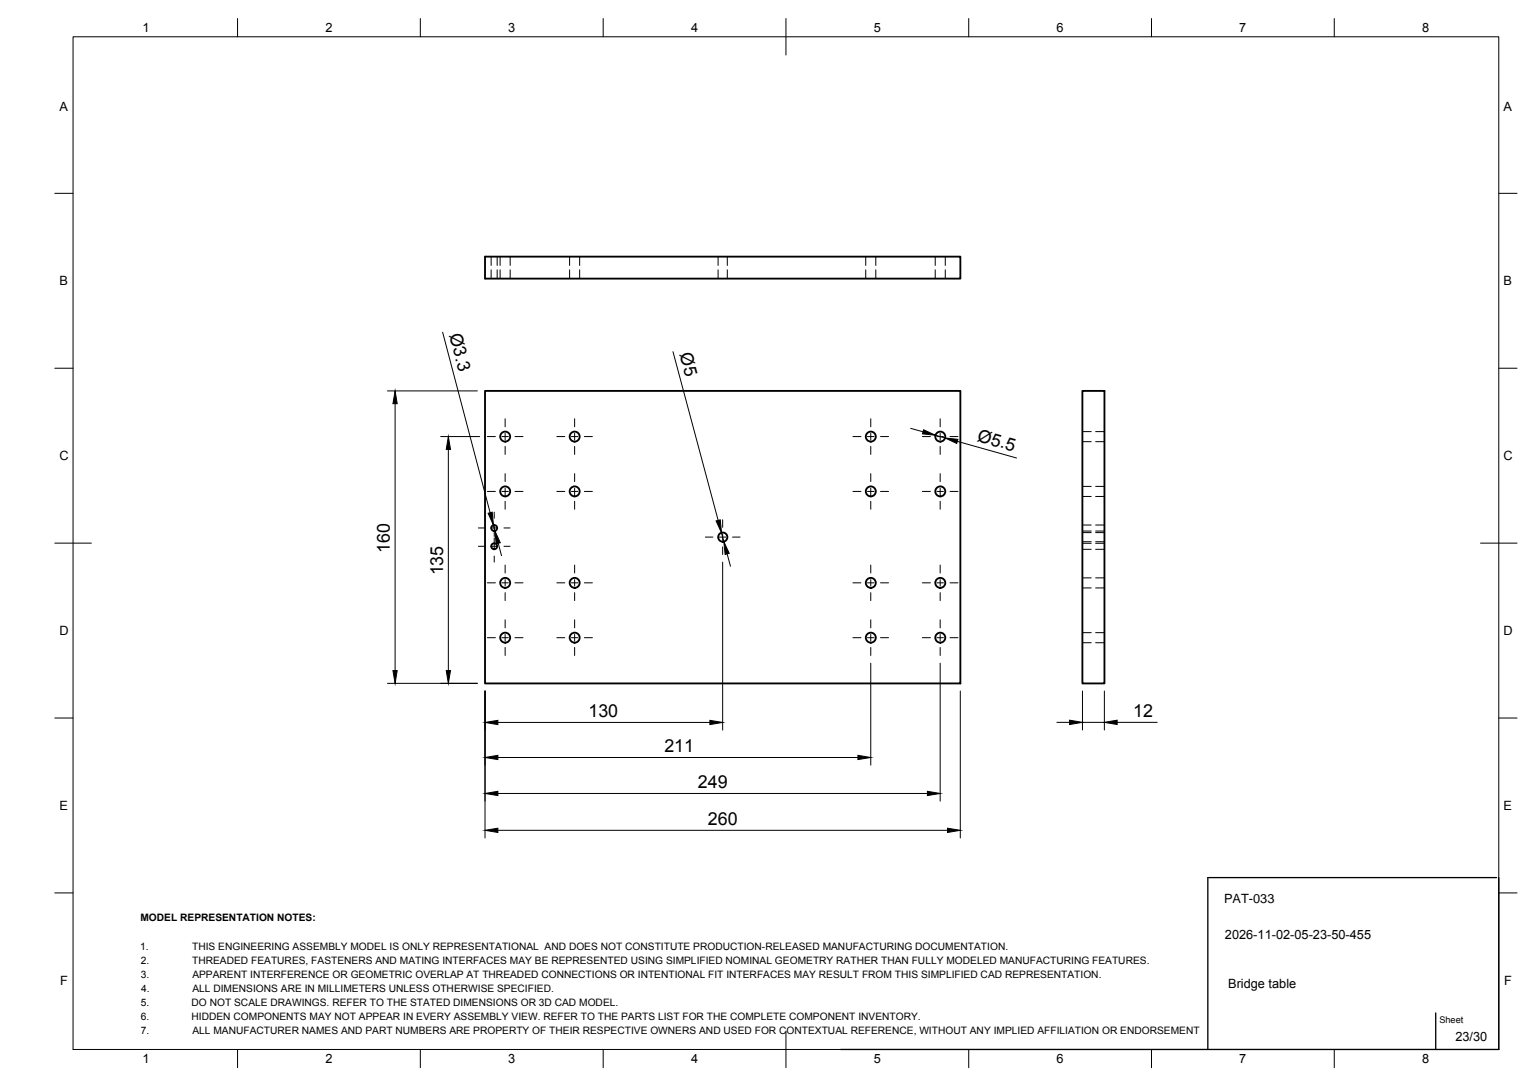
ISO-10303-21;
HEADER;
/* Generated by software containing ST-Developer
 * from STEP Tools, Inc. (www.steptools.com) 
 */

FILE_DESCRIPTION(
/* description */ ('Dual-rail gantry carriage'),
/* implementation_level */ '2;1');

FILE_NAME(
/* name */ 'Bridge table.step',
/* time_stamp */ '2026-10-27T10:49:15-07:00',
/* author */ (''),
/* organization */ (''),
/* preprocessor_version */ 'ST-DEVELOPER v20.2',
/* originating_system */ 'Autodesk Translation Framework v15.17.0.0',
/* authorisation */ '');

FILE_SCHEMA (('AUTOMOTIVE_DESIGN { 1 0 10303 214 3 1 1 }'));
ENDSEC;

DATA;
#10=MECHANICAL_DESIGN_GEOMETRIC_PRESENTATION_REPRESENTATION('',(#604),#12804);
#542=SHAPE_REPRESENTATION_RELATIONSHIP('SRR','None',#13021,#573);
#573=ADVANCED_BREP_SHAPE_REPRESENTATION('',(#633),#12791);
#604=STYLED_ITEM('',(#13233),#633);
#633=MANIFOLD_SOLID_BREP('Body1',#7384);
#707=FACE_BOUND('',#1770,.T.);
#708=FACE_BOUND('',#1771,.T.);
#709=FACE_BOUND('',#1772,.T.);
#710=FACE_BOUND('',#1773,.T.);
#711=FACE_BOUND('',#1774,.T.);
#712=FACE_BOUND('',#1775,.T.);
#713=FACE_BOUND('',#1776,.T.);
#714=FACE_BOUND('',#1777,.T.);
#715=FACE_BOUND('',#1778,.T.);
#716=FACE_BOUND('',#1779,.T.);
#717=FACE_BOUND('',#1780,.T.);
#718=FACE_BOUND('',#1781,.T.);
#719=FACE_BOUND('',#1782,.T.);
#720=FACE_BOUND('',#1783,.T.);
#721=FACE_BOUND('',#1784,.T.);
#722=FACE_BOUND('',#1785,.T.);
#723=FACE_BOUND('',#1786,.T.);
#724=FACE_BOUND('',#1787,.T.);
#725=FACE_BOUND('',#1788,.T.);
#726=FACE_BOUND('',#1790,.T.);
#727=FACE_BOUND('',#1791,.T.);
#728=FACE_BOUND('',#1792,.T.);
#729=FACE_BOUND('',#1793,.T.);
#730=FACE_BOUND('',#1794,.T.);
#731=FACE_BOUND('',#1795,.T.);
#732=FACE_BOUND('',#1796,.T.);
#733=FACE_BOUND('',#1797,.T.);
#734=FACE_BOUND('',#1798,.T.);
#735=FACE_BOUND('',#1799,.T.);
#736=FACE_BOUND('',#1800,.T.);
#737=FACE_BOUND('',#1801,.T.);
#738=FACE_BOUND('',#1802,.T.);
#739=FACE_BOUND('',#1803,.T.);
#740=FACE_BOUND('',#1804,.T.);
#741=FACE_BOUND('',#1805,.T.);
#742=FACE_BOUND('',#1806,.T.);
#743=FACE_BOUND('',#1807,.T.);
#744=FACE_BOUND('',#1808,.T.);
#955=PLANE('',#8168);
#956=PLANE('',#8169);
#957=PLANE('',#8170);
#958=PLANE('',#8171);
#959=PLANE('',#8172);
#960=PLANE('',#8173);
#1292=FACE_OUTER_BOUND('',#1746,.T.);
#1293=FACE_OUTER_BOUND('',#1747,.T.);
#1294=FACE_OUTER_BOUND('',#1748,.T.);
#1295=FACE_OUTER_BOUND('',#1749,.T.);
#1296=FACE_OUTER_BOUND('',#1750,.T.);
#1297=FACE_OUTER_BOUND('',#1751,.T.);
#1298=FACE_OUTER_BOUND('',#1752,.T.);
#1299=FACE_OUTER_BOUND('',#1753,.T.);
#1300=FACE_OUTER_BOUND('',#1754,.T.);
#1301=FACE_OUTER_BOUND('',#1755,.T.);
#1302=FACE_OUTER_BOUND('',#1756,.T.);
#1303=FACE_OUTER_BOUND('',#1757,.T.);
#1304=FACE_OUTER_BOUND('',#1758,.T.);
#1305=FACE_OUTER_BOUND('',#1759,.T.);
#1306=FACE_OUTER_BOUND('',#1760,.T.);
#1307=FACE_OUTER_BOUND('',#1761,.T.);
#1308=FACE_OUTER_BOUND('',#1762,.T.);
#1309=FACE_OUTER_BOUND('',#1763,.T.);
#1310=FACE_OUTER_BOUND('',#1764,.T.);
#1311=FACE_OUTER_BOUND('',#1765,.T.);
#1312=FACE_OUTER_BOUND('',#1766,.T.);
#1313=FACE_OUTER_BOUND('',#1767,.T.);
#1314=FACE_OUTER_BOUND('',#1768,.T.);
#1315=FACE_OUTER_BOUND('',#1769,.T.);
#1316=FACE_OUTER_BOUND('',#1789,.T.);
#1746=EDGE_LOOP('',(#6219,#6220,#6221,#6222));
#1747=EDGE_LOOP('',(#6223,#6224,#6225,#6226));
#1748=EDGE_LOOP('',(#6227,#6228,#6229,#6230));
#1749=EDGE_LOOP('',(#6231,#6232,#6233,#6234));
#1750=EDGE_LOOP('',(#6235,#6236,#6237,#6238));
#1751=EDGE_LOOP('',(#6239,#6240,#6241,#6242));
#1752=EDGE_LOOP('',(#6243,#6244,#6245,#6246));
#1753=EDGE_LOOP('',(#6247,#6248,#6249,#6250));
#1754=EDGE_LOOP('',(#6251,#6252,#6253,#6254));
#1755=EDGE_LOOP('',(#6255,#6256,#6257,#6258));
#1756=EDGE_LOOP('',(#6259,#6260,#6261,#6262));
#1757=EDGE_LOOP('',(#6263,#6264,#6265,#6266));
#1758=EDGE_LOOP('',(#6267,#6268,#6269,#6270));
#1759=EDGE_LOOP('',(#6271,#6272,#6273,#6274));
#1760=EDGE_LOOP('',(#6275,#6276,#6277,#6278));
#1761=EDGE_LOOP('',(#6279,#6280,#6281,#6282));
#1762=EDGE_LOOP('',(#6283,#6284,#6285,#6286));
#1763=EDGE_LOOP('',(#6287,#6288,#6289,#6290));
#1764=EDGE_LOOP('',(#6291,#6292,#6293,#6294));
#1765=EDGE_LOOP('',(#6295,#6296,#6297,#6298));
#1766=EDGE_LOOP('',(#6299,#6300,#6301,#6302));
#1767=EDGE_LOOP('',(#6303,#6304,#6305,#6306));
#1768=EDGE_LOOP('',(#6307,#6308,#6309,#6310));
#1769=EDGE_LOOP('',(#6311,#6312,#6313,#6314));
#1770=EDGE_LOOP('',(#6315));
#1771=EDGE_LOOP('',(#6316));
#1772=EDGE_LOOP('',(#6317));
#1773=EDGE_LOOP('',(#6318));
#1774=EDGE_LOOP('',(#6319));
#1775=EDGE_LOOP('',(#6320));
#1776=EDGE_LOOP('',(#6321));
#1777=EDGE_LOOP('',(#6322));
#1778=EDGE_LOOP('',(#6323));
#1779=EDGE_LOOP('',(#6324));
#1780=EDGE_LOOP('',(#6325));
#1781=EDGE_LOOP('',(#6326));
#1782=EDGE_LOOP('',(#6327));
#1783=EDGE_LOOP('',(#6328));
#1784=EDGE_LOOP('',(#6329));
#1785=EDGE_LOOP('',(#6330));
#1786=EDGE_LOOP('',(#6331));
#1787=EDGE_LOOP('',(#6332));
#1788=EDGE_LOOP('',(#6333));
#1789=EDGE_LOOP('',(#6334,#6335,#6336,#6337));
#1790=EDGE_LOOP('',(#6338));
#1791=EDGE_LOOP('',(#6339));
#1792=EDGE_LOOP('',(#6340));
#1793=EDGE_LOOP('',(#6341));
#1794=EDGE_LOOP('',(#6342));
#1795=EDGE_LOOP('',(#6343));
#1796=EDGE_LOOP('',(#6344));
#1797=EDGE_LOOP('',(#6345));
#1798=EDGE_LOOP('',(#6346));
#1799=EDGE_LOOP('',(#6347));
#1800=EDGE_LOOP('',(#6348));
#1801=EDGE_LOOP('',(#6349));
#1802=EDGE_LOOP('',(#6350));
#1803=EDGE_LOOP('',(#6351));
#1804=EDGE_LOOP('',(#6352));
#1805=EDGE_LOOP('',(#6353));
#1806=EDGE_LOOP('',(#6354));
#1807=EDGE_LOOP('',(#6355));
#1808=EDGE_LOOP('',(#6356));
#2421=LINE('',#11906,#3130);
#2422=LINE('',#11912,#3131);
#2423=LINE('',#11918,#3132);
#2424=LINE('',#11924,#3133);
#2425=LINE('',#11930,#3134);
#2426=LINE('',#11936,#3135);
#2427=LINE('',#11942,#3136);
#2428=LINE('',#11948,#3137);
#2429=LINE('',#11954,#3138);
#2430=LINE('',#11960,#3139);
#2431=LINE('',#11966,#3140);
#2432=LINE('',#11972,#3141);
#2433=LINE('',#11978,#3142);
#2434=LINE('',#11984,#3143);
#2435=LINE('',#11990,#3144);
#2436=LINE('',#11996,#3145);
#2437=LINE('',#12002,#3146);
#2438=LINE('',#12008,#3147);
#2439=LINE('',#12014,#3148);
#2440=LINE('',#12019,#3149);
#2441=LINE('',#12021,#3150);
#2442=LINE('',#12023,#3151);
#2443=LINE('',#12024,#3152);
#2444=LINE('',#12027,#3153);
#2445=LINE('',#12029,#3154);
#2446=LINE('',#12030,#3155);
#2447=LINE('',#12033,#3156);
#2448=LINE('',#12035,#3157);
#2449=LINE('',#12036,#3158);
#2450=LINE('',#12038,#3159);
#2451=LINE('',#12039,#3160);
#3130=VECTOR('',#9704,0.164999999999999);
#3131=VECTOR('',#9711,0.164999999999999);
#3132=VECTOR('',#9718,0.25);
#3133=VECTOR('',#9725,0.274999999999999);
#3134=VECTOR('',#9732,0.274999999999999);
#3135=VECTOR('',#9739,0.274999999999999);
#3136=VECTOR('',#9746,0.274999999999999);
#3137=VECTOR('',#9753,0.274999999999999);
#3138=VECTOR('',#9760,0.275);
#3139=VECTOR('',#9767,0.275);
#3140=VECTOR('',#9774,0.274999999999999);
#3141=VECTOR('',#9781,0.274999999999999);
#3142=VECTOR('',#9788,0.274999999999999);
#3143=VECTOR('',#9795,0.274999999999999);
#3144=VECTOR('',#9802,0.274999999999999);
#3145=VECTOR('',#9809,0.274999999999999);
#3146=VECTOR('',#9816,0.275);
#3147=VECTOR('',#9823,0.275);
#3148=VECTOR('',#9830,0.274999999999999);
#3149=VECTOR('',#9835,1.);
#3150=VECTOR('',#9836,1.);
#3151=VECTOR('',#9837,1.);
#3152=VECTOR('',#9838,1.);
#3153=VECTOR('',#9841,1.);
#3154=VECTOR('',#9842,1.);
#3155=VECTOR('',#9843,1.);
#3156=VECTOR('',#9846,1.);
#3157=VECTOR('',#9847,1.);
#3158=VECTOR('',#9848,1.);
#3159=VECTOR('',#9851,1.);
#3160=VECTOR('',#9852,1.);
#3467=CIRCLE('',#8112,0.164999999999999);
#3468=CIRCLE('',#8113,0.164999999999999);
#3469=CIRCLE('',#8115,0.164999999999999);
#3470=CIRCLE('',#8116,0.164999999999999);
#3471=CIRCLE('',#8118,0.25);
#3472=CIRCLE('',#8119,0.25);
#3473=CIRCLE('',#8121,0.274999999999999);
#3474=CIRCLE('',#8122,0.274999999999999);
#3475=CIRCLE('',#8124,0.274999999999999);
#3476=CIRCLE('',#8125,0.274999999999999);
#3477=CIRCLE('',#8127,0.274999999999999);
#3478=CIRCLE('',#8128,0.274999999999999);
#3479=CIRCLE('',#8130,0.274999999999999);
#3480=CIRCLE('',#8131,0.274999999999999);
#3481=CIRCLE('',#8133,0.274999999999999);
#3482=CIRCLE('',#8134,0.274999999999999);
#3483=CIRCLE('',#8136,0.275);
#3484=CIRCLE('',#8137,0.275);
#3485=CIRCLE('',#8139,0.275);
#3486=CIRCLE('',#8140,0.275);
#3487=CIRCLE('',#8142,0.274999999999999);
#3488=CIRCLE('',#8143,0.274999999999999);
#3489=CIRCLE('',#8145,0.274999999999999);
#3490=CIRCLE('',#8146,0.274999999999999);
#3491=CIRCLE('',#8148,0.274999999999999);
#3492=CIRCLE('',#8149,0.274999999999999);
#3493=CIRCLE('',#8151,0.274999999999999);
#3494=CIRCLE('',#8152,0.274999999999999);
#3495=CIRCLE('',#8154,0.274999999999999);
#3496=CIRCLE('',#8155,0.274999999999999);
#3497=CIRCLE('',#8157,0.274999999999999);
#3498=CIRCLE('',#8158,0.274999999999999);
#3499=CIRCLE('',#8160,0.275);
#3500=CIRCLE('',#8161,0.275);
#3501=CIRCLE('',#8163,0.275);
#3502=CIRCLE('',#8164,0.275);
#3503=CIRCLE('',#8166,0.274999999999999);
#3504=CIRCLE('',#8167,0.274999999999999);
#3937=VERTEX_POINT('',#11903);
#3938=VERTEX_POINT('',#11905);
#3939=VERTEX_POINT('',#11909);
#3940=VERTEX_POINT('',#11911);
#3941=VERTEX_POINT('',#11915);
#3942=VERTEX_POINT('',#11917);
#3943=VERTEX_POINT('',#11921);
#3944=VERTEX_POINT('',#11923);
#3945=VERTEX_POINT('',#11927);
#3946=VERTEX_POINT('',#11929);
#3947=VERTEX_POINT('',#11933);
#3948=VERTEX_POINT('',#11935);
#3949=VERTEX_POINT('',#11939);
#3950=VERTEX_POINT('',#11941);
#3951=VERTEX_POINT('',#11945);
#3952=VERTEX_POINT('',#11947);
#3953=VERTEX_POINT('',#11951);
#3954=VERTEX_POINT('',#11953);
#3955=VERTEX_POINT('',#11957);
#3956=VERTEX_POINT('',#11959);
#3957=VERTEX_POINT('',#11963);
#3958=VERTEX_POINT('',#11965);
#3959=VERTEX_POINT('',#11969);
#3960=VERTEX_POINT('',#11971);
#3961=VERTEX_POINT('',#11975);
#3962=VERTEX_POINT('',#11977);
#3963=VERTEX_POINT('',#11981);
#3964=VERTEX_POINT('',#11983);
#3965=VERTEX_POINT('',#11987);
#3966=VERTEX_POINT('',#11989);
#3967=VERTEX_POINT('',#11993);
#3968=VERTEX_POINT('',#11995);
#3969=VERTEX_POINT('',#11999);
#3970=VERTEX_POINT('',#12001);
#3971=VERTEX_POINT('',#12005);
#3972=VERTEX_POINT('',#12007);
#3973=VERTEX_POINT('',#12011);
#3974=VERTEX_POINT('',#12013);
#3975=VERTEX_POINT('',#12017);
#3976=VERTEX_POINT('',#12018);
#3977=VERTEX_POINT('',#12020);
#3978=VERTEX_POINT('',#12022);
#3979=VERTEX_POINT('',#12026);
#3980=VERTEX_POINT('',#12028);
#3981=VERTEX_POINT('',#12032);
#3982=VERTEX_POINT('',#12034);
#4732=EDGE_CURVE('',#3937,#3937,#3467,.T.);
#4733=EDGE_CURVE('',#3937,#3938,#2421,.T.);
#4734=EDGE_CURVE('',#3938,#3938,#3468,.T.);
#4735=EDGE_CURVE('',#3939,#3939,#3469,.T.);
#4736=EDGE_CURVE('',#3939,#3940,#2422,.T.);
#4737=EDGE_CURVE('',#3940,#3940,#3470,.T.);
#4738=EDGE_CURVE('',#3941,#3941,#3471,.T.);
#4739=EDGE_CURVE('',#3941,#3942,#2423,.T.);
#4740=EDGE_CURVE('',#3942,#3942,#3472,.T.);
#4741=EDGE_CURVE('',#3943,#3943,#3473,.T.);
#4742=EDGE_CURVE('',#3943,#3944,#2424,.T.);
#4743=EDGE_CURVE('',#3944,#3944,#3474,.T.);
#4744=EDGE_CURVE('',#3945,#3945,#3475,.T.);
#4745=EDGE_CURVE('',#3945,#3946,#2425,.T.);
#4746=EDGE_CURVE('',#3946,#3946,#3476,.T.);
#4747=EDGE_CURVE('',#3947,#3947,#3477,.T.);
#4748=EDGE_CURVE('',#3947,#3948,#2426,.T.);
#4749=EDGE_CURVE('',#3948,#3948,#3478,.T.);
#4750=EDGE_CURVE('',#3949,#3949,#3479,.T.);
#4751=EDGE_CURVE('',#3949,#3950,#2427,.T.);
#4752=EDGE_CURVE('',#3950,#3950,#3480,.T.);
#4753=EDGE_CURVE('',#3951,#3951,#3481,.T.);
#4754=EDGE_CURVE('',#3951,#3952,#2428,.T.);
#4755=EDGE_CURVE('',#3952,#3952,#3482,.T.);
#4756=EDGE_CURVE('',#3953,#3953,#3483,.T.);
#4757=EDGE_CURVE('',#3953,#3954,#2429,.T.);
#4758=EDGE_CURVE('',#3954,#3954,#3484,.T.);
#4759=EDGE_CURVE('',#3955,#3955,#3485,.T.);
#4760=EDGE_CURVE('',#3955,#3956,#2430,.T.);
#4761=EDGE_CURVE('',#3956,#3956,#3486,.T.);
#4762=EDGE_CURVE('',#3957,#3957,#3487,.T.);
#4763=EDGE_CURVE('',#3957,#3958,#2431,.T.);
#4764=EDGE_CURVE('',#3958,#3958,#3488,.T.);
#4765=EDGE_CURVE('',#3959,#3959,#3489,.T.);
#4766=EDGE_CURVE('',#3959,#3960,#2432,.T.);
#4767=EDGE_CURVE('',#3960,#3960,#3490,.T.);
#4768=EDGE_CURVE('',#3961,#3961,#3491,.T.);
#4769=EDGE_CURVE('',#3961,#3962,#2433,.T.);
#4770=EDGE_CURVE('',#3962,#3962,#3492,.T.);
#4771=EDGE_CURVE('',#3963,#3963,#3493,.T.);
#4772=EDGE_CURVE('',#3963,#3964,#2434,.T.);
#4773=EDGE_CURVE('',#3964,#3964,#3494,.T.);
#4774=EDGE_CURVE('',#3965,#3965,#3495,.T.);
#4775=EDGE_CURVE('',#3965,#3966,#2435,.T.);
#4776=EDGE_CURVE('',#3966,#3966,#3496,.T.);
#4777=EDGE_CURVE('',#3967,#3967,#3497,.T.);
#4778=EDGE_CURVE('',#3967,#3968,#2436,.T.);
#4779=EDGE_CURVE('',#3968,#3968,#3498,.T.);
#4780=EDGE_CURVE('',#3969,#3969,#3499,.T.);
#4781=EDGE_CURVE('',#3969,#3970,#2437,.T.);
#4782=EDGE_CURVE('',#3970,#3970,#3500,.T.);
#4783=EDGE_CURVE('',#3971,#3971,#3501,.T.);
#4784=EDGE_CURVE('',#3971,#3972,#2438,.T.);
#4785=EDGE_CURVE('',#3972,#3972,#3502,.T.);
#4786=EDGE_CURVE('',#3973,#3973,#3503,.T.);
#4787=EDGE_CURVE('',#3973,#3974,#2439,.T.);
#4788=EDGE_CURVE('',#3974,#3974,#3504,.T.);
#4789=EDGE_CURVE('',#3975,#3976,#2440,.T.);
#4790=EDGE_CURVE('',#3976,#3977,#2441,.T.);
#4791=EDGE_CURVE('',#3978,#3977,#2442,.T.);
#4792=EDGE_CURVE('',#3975,#3978,#2443,.T.);
#4793=EDGE_CURVE('',#3979,#3975,#2444,.T.);
#4794=EDGE_CURVE('',#3980,#3978,#2445,.T.);
#4795=EDGE_CURVE('',#3979,#3980,#2446,.T.);
#4796=EDGE_CURVE('',#3981,#3979,#2447,.T.);
#4797=EDGE_CURVE('',#3982,#3980,#2448,.T.);
#4798=EDGE_CURVE('',#3981,#3982,#2449,.T.);
#4799=EDGE_CURVE('',#3976,#3981,#2450,.T.);
#4800=EDGE_CURVE('',#3977,#3982,#2451,.T.);
#6219=ORIENTED_EDGE('',*,*,#4732,.F.);
#6220=ORIENTED_EDGE('',*,*,#4733,.T.);
#6221=ORIENTED_EDGE('',*,*,#4734,.F.);
#6222=ORIENTED_EDGE('',*,*,#4733,.F.);
#6223=ORIENTED_EDGE('',*,*,#4735,.F.);
#6224=ORIENTED_EDGE('',*,*,#4736,.T.);
#6225=ORIENTED_EDGE('',*,*,#4737,.F.);
#6226=ORIENTED_EDGE('',*,*,#4736,.F.);
#6227=ORIENTED_EDGE('',*,*,#4738,.F.);
#6228=ORIENTED_EDGE('',*,*,#4739,.T.);
#6229=ORIENTED_EDGE('',*,*,#4740,.F.);
#6230=ORIENTED_EDGE('',*,*,#4739,.F.);
#6231=ORIENTED_EDGE('',*,*,#4741,.F.);
#6232=ORIENTED_EDGE('',*,*,#4742,.T.);
#6233=ORIENTED_EDGE('',*,*,#4743,.F.);
#6234=ORIENTED_EDGE('',*,*,#4742,.F.);
#6235=ORIENTED_EDGE('',*,*,#4744,.F.);
#6236=ORIENTED_EDGE('',*,*,#4745,.T.);
#6237=ORIENTED_EDGE('',*,*,#4746,.F.);
#6238=ORIENTED_EDGE('',*,*,#4745,.F.);
#6239=ORIENTED_EDGE('',*,*,#4747,.F.);
#6240=ORIENTED_EDGE('',*,*,#4748,.T.);
#6241=ORIENTED_EDGE('',*,*,#4749,.F.);
#6242=ORIENTED_EDGE('',*,*,#4748,.F.);
#6243=ORIENTED_EDGE('',*,*,#4750,.F.);
#6244=ORIENTED_EDGE('',*,*,#4751,.T.);
#6245=ORIENTED_EDGE('',*,*,#4752,.F.);
#6246=ORIENTED_EDGE('',*,*,#4751,.F.);
#6247=ORIENTED_EDGE('',*,*,#4753,.F.);
#6248=ORIENTED_EDGE('',*,*,#4754,.T.);
#6249=ORIENTED_EDGE('',*,*,#4755,.F.);
#6250=ORIENTED_EDGE('',*,*,#4754,.F.);
#6251=ORIENTED_EDGE('',*,*,#4756,.F.);
#6252=ORIENTED_EDGE('',*,*,#4757,.T.);
#6253=ORIENTED_EDGE('',*,*,#4758,.F.);
#6254=ORIENTED_EDGE('',*,*,#4757,.F.);
#6255=ORIENTED_EDGE('',*,*,#4759,.F.);
#6256=ORIENTED_EDGE('',*,*,#4760,.T.);
#6257=ORIENTED_EDGE('',*,*,#4761,.F.);
#6258=ORIENTED_EDGE('',*,*,#4760,.F.);
#6259=ORIENTED_EDGE('',*,*,#4762,.F.);
#6260=ORIENTED_EDGE('',*,*,#4763,.T.);
#6261=ORIENTED_EDGE('',*,*,#4764,.F.);
#6262=ORIENTED_EDGE('',*,*,#4763,.F.);
#6263=ORIENTED_EDGE('',*,*,#4765,.F.);
#6264=ORIENTED_EDGE('',*,*,#4766,.T.);
#6265=ORIENTED_EDGE('',*,*,#4767,.F.);
#6266=ORIENTED_EDGE('',*,*,#4766,.F.);
#6267=ORIENTED_EDGE('',*,*,#4768,.F.);
#6268=ORIENTED_EDGE('',*,*,#4769,.T.);
#6269=ORIENTED_EDGE('',*,*,#4770,.F.);
#6270=ORIENTED_EDGE('',*,*,#4769,.F.);
#6271=ORIENTED_EDGE('',*,*,#4771,.F.);
#6272=ORIENTED_EDGE('',*,*,#4772,.T.);
#6273=ORIENTED_EDGE('',*,*,#4773,.F.);
#6274=ORIENTED_EDGE('',*,*,#4772,.F.);
#6275=ORIENTED_EDGE('',*,*,#4774,.F.);
#6276=ORIENTED_EDGE('',*,*,#4775,.T.);
#6277=ORIENTED_EDGE('',*,*,#4776,.F.);
#6278=ORIENTED_EDGE('',*,*,#4775,.F.);
#6279=ORIENTED_EDGE('',*,*,#4777,.F.);
#6280=ORIENTED_EDGE('',*,*,#4778,.T.);
#6281=ORIENTED_EDGE('',*,*,#4779,.F.);
#6282=ORIENTED_EDGE('',*,*,#4778,.F.);
#6283=ORIENTED_EDGE('',*,*,#4780,.F.);
#6284=ORIENTED_EDGE('',*,*,#4781,.T.);
#6285=ORIENTED_EDGE('',*,*,#4782,.F.);
#6286=ORIENTED_EDGE('',*,*,#4781,.F.);
#6287=ORIENTED_EDGE('',*,*,#4783,.F.);
#6288=ORIENTED_EDGE('',*,*,#4784,.T.);
#6289=ORIENTED_EDGE('',*,*,#4785,.F.);
#6290=ORIENTED_EDGE('',*,*,#4784,.F.);
#6291=ORIENTED_EDGE('',*,*,#4786,.F.);
#6292=ORIENTED_EDGE('',*,*,#4787,.T.);
#6293=ORIENTED_EDGE('',*,*,#4788,.F.);
#6294=ORIENTED_EDGE('',*,*,#4787,.F.);
#6295=ORIENTED_EDGE('',*,*,#4789,.T.);
#6296=ORIENTED_EDGE('',*,*,#4790,.T.);
#6297=ORIENTED_EDGE('',*,*,#4791,.F.);
#6298=ORIENTED_EDGE('',*,*,#4792,.F.);
#6299=ORIENTED_EDGE('',*,*,#4793,.T.);
#6300=ORIENTED_EDGE('',*,*,#4792,.T.);
#6301=ORIENTED_EDGE('',*,*,#4794,.F.);
#6302=ORIENTED_EDGE('',*,*,#4795,.F.);
#6303=ORIENTED_EDGE('',*,*,#4796,.T.);
#6304=ORIENTED_EDGE('',*,*,#4795,.T.);
#6305=ORIENTED_EDGE('',*,*,#4797,.F.);
#6306=ORIENTED_EDGE('',*,*,#4798,.F.);
#6307=ORIENTED_EDGE('',*,*,#4799,.T.);
#6308=ORIENTED_EDGE('',*,*,#4798,.T.);
#6309=ORIENTED_EDGE('',*,*,#4800,.F.);
#6310=ORIENTED_EDGE('',*,*,#4790,.F.);
#6311=ORIENTED_EDGE('',*,*,#4800,.T.);
#6312=ORIENTED_EDGE('',*,*,#4797,.T.);
#6313=ORIENTED_EDGE('',*,*,#4794,.T.);
#6314=ORIENTED_EDGE('',*,*,#4791,.T.);
#6315=ORIENTED_EDGE('',*,*,#4740,.T.);
#6316=ORIENTED_EDGE('',*,*,#4755,.T.);
#6317=ORIENTED_EDGE('',*,*,#4758,.T.);
#6318=ORIENTED_EDGE('',*,*,#4761,.T.);
#6319=ORIENTED_EDGE('',*,*,#4764,.T.);
#6320=ORIENTED_EDGE('',*,*,#4788,.T.);
#6321=ORIENTED_EDGE('',*,*,#4785,.T.);
#6322=ORIENTED_EDGE('',*,*,#4782,.T.);
#6323=ORIENTED_EDGE('',*,*,#4779,.T.);
#6324=ORIENTED_EDGE('',*,*,#4776,.T.);
#6325=ORIENTED_EDGE('',*,*,#4773,.T.);
#6326=ORIENTED_EDGE('',*,*,#4770,.T.);
#6327=ORIENTED_EDGE('',*,*,#4767,.T.);
#6328=ORIENTED_EDGE('',*,*,#4752,.T.);
#6329=ORIENTED_EDGE('',*,*,#4749,.T.);
#6330=ORIENTED_EDGE('',*,*,#4746,.T.);
#6331=ORIENTED_EDGE('',*,*,#4743,.T.);
#6332=ORIENTED_EDGE('',*,*,#4737,.T.);
#6333=ORIENTED_EDGE('',*,*,#4734,.T.);
#6334=ORIENTED_EDGE('',*,*,#4799,.F.);
#6335=ORIENTED_EDGE('',*,*,#4789,.F.);
#6336=ORIENTED_EDGE('',*,*,#4793,.F.);
#6337=ORIENTED_EDGE('',*,*,#4796,.F.);
#6338=ORIENTED_EDGE('',*,*,#4738,.T.);
#6339=ORIENTED_EDGE('',*,*,#4753,.T.);
#6340=ORIENTED_EDGE('',*,*,#4756,.T.);
#6341=ORIENTED_EDGE('',*,*,#4759,.T.);
#6342=ORIENTED_EDGE('',*,*,#4762,.T.);
#6343=ORIENTED_EDGE('',*,*,#4786,.T.);
#6344=ORIENTED_EDGE('',*,*,#4783,.T.);
#6345=ORIENTED_EDGE('',*,*,#4780,.T.);
#6346=ORIENTED_EDGE('',*,*,#4777,.T.);
#6347=ORIENTED_EDGE('',*,*,#4774,.T.);
#6348=ORIENTED_EDGE('',*,*,#4771,.T.);
#6349=ORIENTED_EDGE('',*,*,#4768,.T.);
#6350=ORIENTED_EDGE('',*,*,#4765,.T.);
#6351=ORIENTED_EDGE('',*,*,#4750,.T.);
#6352=ORIENTED_EDGE('',*,*,#4747,.T.);
#6353=ORIENTED_EDGE('',*,*,#4744,.T.);
#6354=ORIENTED_EDGE('',*,*,#4741,.T.);
#6355=ORIENTED_EDGE('',*,*,#4735,.T.);
#6356=ORIENTED_EDGE('',*,*,#4732,.T.);
#6935=CYLINDRICAL_SURFACE('',#8111,0.164999999999999);
#6936=CYLINDRICAL_SURFACE('',#8114,0.164999999999999);
#6937=CYLINDRICAL_SURFACE('',#8117,0.25);
#6938=CYLINDRICAL_SURFACE('',#8120,0.274999999999999);
#6939=CYLINDRICAL_SURFACE('',#8123,0.274999999999999);
#6940=CYLINDRICAL_SURFACE('',#8126,0.274999999999999);
#6941=CYLINDRICAL_SURFACE('',#8129,0.274999999999999);
#6942=CYLINDRICAL_SURFACE('',#8132,0.274999999999999);
#6943=CYLINDRICAL_SURFACE('',#8135,0.275);
#6944=CYLINDRICAL_SURFACE('',#8138,0.275);
#6945=CYLINDRICAL_SURFACE('',#8141,0.274999999999999);
#6946=CYLINDRICAL_SURFACE('',#8144,0.274999999999999);
#6947=CYLINDRICAL_SURFACE('',#8147,0.274999999999999);
#6948=CYLINDRICAL_SURFACE('',#8150,0.274999999999999);
#6949=CYLINDRICAL_SURFACE('',#8153,0.274999999999999);
#6950=CYLINDRICAL_SURFACE('',#8156,0.274999999999999);
#6951=CYLINDRICAL_SURFACE('',#8159,0.275);
#6952=CYLINDRICAL_SURFACE('',#8162,0.275);
#6953=CYLINDRICAL_SURFACE('',#8165,0.274999999999999);
#7218=ADVANCED_FACE('',(#1292),#6935,.F.);
#7219=ADVANCED_FACE('',(#1293),#6936,.F.);
#7220=ADVANCED_FACE('',(#1294),#6937,.F.);
#7221=ADVANCED_FACE('',(#1295),#6938,.F.);
#7222=ADVANCED_FACE('',(#1296),#6939,.F.);
#7223=ADVANCED_FACE('',(#1297),#6940,.F.);
#7224=ADVANCED_FACE('',(#1298),#6941,.F.);
#7225=ADVANCED_FACE('',(#1299),#6942,.F.);
#7226=ADVANCED_FACE('',(#1300),#6943,.F.);
#7227=ADVANCED_FACE('',(#1301),#6944,.F.);
#7228=ADVANCED_FACE('',(#1302),#6945,.F.);
#7229=ADVANCED_FACE('',(#1303),#6946,.F.);
#7230=ADVANCED_FACE('',(#1304),#6947,.F.);
#7231=ADVANCED_FACE('',(#1305),#6948,.F.);
#7232=ADVANCED_FACE('',(#1306),#6949,.F.);
#7233=ADVANCED_FACE('',(#1307),#6950,.F.);
#7234=ADVANCED_FACE('',(#1308),#6951,.F.);
#7235=ADVANCED_FACE('',(#1309),#6952,.F.);
#7236=ADVANCED_FACE('',(#1310),#6953,.F.);
#7237=ADVANCED_FACE('',(#1311),#955,.T.);
#7238=ADVANCED_FACE('',(#1312),#956,.T.);
#7239=ADVANCED_FACE('',(#1313),#957,.T.);
#7240=ADVANCED_FACE('',(#1314),#958,.T.);
#7241=ADVANCED_FACE('',(#1315,#707,#708,#709,#710,#711,#712,#713,#714,#715,
#716,#717,#718,#719,#720,#721,#722,#723,#724,#725),#959,.T.);
#7242=ADVANCED_FACE('',(#1316,#726,#727,#728,#729,#730,#731,#732,#733,#734,
#735,#736,#737,#738,#739,#740,#741,#742,#743,#744),#960,.F.);
#7384=CLOSED_SHELL('',(#7218,#7219,#7220,#7221,#7222,#7223,#7224,#7225,
#7226,#7227,#7228,#7229,#7230,#7231,#7232,#7233,#7234,#7235,#7236,#7237,
#7238,#7239,#7240,#7241,#7242));
#8110=AXIS2_PLACEMENT_3D('',#11901,#9698,#9699);
#8111=AXIS2_PLACEMENT_3D('',#11902,#9700,#9701);
#8112=AXIS2_PLACEMENT_3D('',#11904,#9702,#9703);
#8113=AXIS2_PLACEMENT_3D('',#11907,#9705,#9706);
#8114=AXIS2_PLACEMENT_3D('',#11908,#9707,#9708);
#8115=AXIS2_PLACEMENT_3D('',#11910,#9709,#9710);
#8116=AXIS2_PLACEMENT_3D('',#11913,#9712,#9713);
#8117=AXIS2_PLACEMENT_3D('',#11914,#9714,#9715);
#8118=AXIS2_PLACEMENT_3D('',#11916,#9716,#9717);
#8119=AXIS2_PLACEMENT_3D('',#11919,#9719,#9720);
#8120=AXIS2_PLACEMENT_3D('',#11920,#9721,#9722);
#8121=AXIS2_PLACEMENT_3D('',#11922,#9723,#9724);
#8122=AXIS2_PLACEMENT_3D('',#11925,#9726,#9727);
#8123=AXIS2_PLACEMENT_3D('',#11926,#9728,#9729);
#8124=AXIS2_PLACEMENT_3D('',#11928,#9730,#9731);
#8125=AXIS2_PLACEMENT_3D('',#11931,#9733,#9734);
#8126=AXIS2_PLACEMENT_3D('',#11932,#9735,#9736);
#8127=AXIS2_PLACEMENT_3D('',#11934,#9737,#9738);
#8128=AXIS2_PLACEMENT_3D('',#11937,#9740,#9741);
#8129=AXIS2_PLACEMENT_3D('',#11938,#9742,#9743);
#8130=AXIS2_PLACEMENT_3D('',#11940,#9744,#9745);
#8131=AXIS2_PLACEMENT_3D('',#11943,#9747,#9748);
#8132=AXIS2_PLACEMENT_3D('',#11944,#9749,#9750);
#8133=AXIS2_PLACEMENT_3D('',#11946,#9751,#9752);
#8134=AXIS2_PLACEMENT_3D('',#11949,#9754,#9755);
#8135=AXIS2_PLACEMENT_3D('',#11950,#9756,#9757);
#8136=AXIS2_PLACEMENT_3D('',#11952,#9758,#9759);
#8137=AXIS2_PLACEMENT_3D('',#11955,#9761,#9762);
#8138=AXIS2_PLACEMENT_3D('',#11956,#9763,#9764);
#8139=AXIS2_PLACEMENT_3D('',#11958,#9765,#9766);
#8140=AXIS2_PLACEMENT_3D('',#11961,#9768,#9769);
#8141=AXIS2_PLACEMENT_3D('',#11962,#9770,#9771);
#8142=AXIS2_PLACEMENT_3D('',#11964,#9772,#9773);
#8143=AXIS2_PLACEMENT_3D('',#11967,#9775,#9776);
#8144=AXIS2_PLACEMENT_3D('',#11968,#9777,#9778);
#8145=AXIS2_PLACEMENT_3D('',#11970,#9779,#9780);
#8146=AXIS2_PLACEMENT_3D('',#11973,#9782,#9783);
#8147=AXIS2_PLACEMENT_3D('',#11974,#9784,#9785);
#8148=AXIS2_PLACEMENT_3D('',#11976,#9786,#9787);
#8149=AXIS2_PLACEMENT_3D('',#11979,#9789,#9790);
#8150=AXIS2_PLACEMENT_3D('',#11980,#9791,#9792);
#8151=AXIS2_PLACEMENT_3D('',#11982,#9793,#9794);
#8152=AXIS2_PLACEMENT_3D('',#11985,#9796,#9797);
#8153=AXIS2_PLACEMENT_3D('',#11986,#9798,#9799);
#8154=AXIS2_PLACEMENT_3D('',#11988,#9800,#9801);
#8155=AXIS2_PLACEMENT_3D('',#11991,#9803,#9804);
#8156=AXIS2_PLACEMENT_3D('',#11992,#9805,#9806);
#8157=AXIS2_PLACEMENT_3D('',#11994,#9807,#9808);
#8158=AXIS2_PLACEMENT_3D('',#11997,#9810,#9811);
#8159=AXIS2_PLACEMENT_3D('',#11998,#9812,#9813);
#8160=AXIS2_PLACEMENT_3D('',#12000,#9814,#9815);
#8161=AXIS2_PLACEMENT_3D('',#12003,#9817,#9818);
#8162=AXIS2_PLACEMENT_3D('',#12004,#9819,#9820);
#8163=AXIS2_PLACEMENT_3D('',#12006,#9821,#9822);
#8164=AXIS2_PLACEMENT_3D('',#12009,#9824,#9825);
#8165=AXIS2_PLACEMENT_3D('',#12010,#9826,#9827);
#8166=AXIS2_PLACEMENT_3D('',#12012,#9828,#9829);
#8167=AXIS2_PLACEMENT_3D('',#12015,#9831,#9832);
#8168=AXIS2_PLACEMENT_3D('',#12016,#9833,#9834);
#8169=AXIS2_PLACEMENT_3D('',#12025,#9839,#9840);
#8170=AXIS2_PLACEMENT_3D('',#12031,#9844,#9845);
#8171=AXIS2_PLACEMENT_3D('',#12037,#9849,#9850);
#8172=AXIS2_PLACEMENT_3D('',#12040,#9853,#9854);
#8173=AXIS2_PLACEMENT_3D('',#12041,#9855,#9856);
#9698=DIRECTION('axis',(0.,0.,1.));
#9699=DIRECTION('refdir',(1.,0.,0.));
#9700=DIRECTION('center_axis',(0.,0.,1.));
#9701=DIRECTION('ref_axis',(1.,0.,0.));
#9702=DIRECTION('center_axis',(0.,0.,1.));
#9703=DIRECTION('ref_axis',(1.,0.,0.));
#9704=DIRECTION('',(0.,0.,1.));
#9705=DIRECTION('center_axis',(0.,0.,-1.));
#9706=DIRECTION('ref_axis',(1.,0.,0.));
#9707=DIRECTION('center_axis',(0.,0.,1.));
#9708=DIRECTION('ref_axis',(1.,0.,0.));
#9709=DIRECTION('center_axis',(0.,0.,1.));
#9710=DIRECTION('ref_axis',(1.,0.,0.));
#9711=DIRECTION('',(0.,0.,1.));
#9712=DIRECTION('center_axis',(0.,0.,-1.));
#9713=DIRECTION('ref_axis',(1.,0.,0.));
#9714=DIRECTION('center_axis',(0.,0.,1.));
#9715=DIRECTION('ref_axis',(1.,0.,0.));
#9716=DIRECTION('center_axis',(0.,0.,1.));
#9717=DIRECTION('ref_axis',(1.,0.,0.));
#9718=DIRECTION('',(0.,0.,1.));
#9719=DIRECTION('center_axis',(0.,0.,-1.));
#9720=DIRECTION('ref_axis',(1.,0.,0.));
#9721=DIRECTION('center_axis',(0.,0.,1.));
#9722=DIRECTION('ref_axis',(1.,0.,0.));
#9723=DIRECTION('center_axis',(0.,0.,1.));
#9724=DIRECTION('ref_axis',(1.,0.,0.));
#9725=DIRECTION('',(0.,0.,1.));
#9726=DIRECTION('center_axis',(0.,0.,-1.));
#9727=DIRECTION('ref_axis',(1.,0.,0.));
#9728=DIRECTION('center_axis',(0.,0.,1.));
#9729=DIRECTION('ref_axis',(1.,0.,0.));
#9730=DIRECTION('center_axis',(0.,0.,1.));
#9731=DIRECTION('ref_axis',(1.,0.,0.));
#9732=DIRECTION('',(0.,0.,1.));
#9733=DIRECTION('center_axis',(0.,0.,-1.));
#9734=DIRECTION('ref_axis',(1.,0.,0.));
#9735=DIRECTION('center_axis',(0.,0.,1.));
#9736=DIRECTION('ref_axis',(1.,0.,0.));
#9737=DIRECTION('center_axis',(0.,0.,1.));
#9738=DIRECTION('ref_axis',(1.,0.,0.));
#9739=DIRECTION('',(0.,0.,1.));
#9740=DIRECTION('center_axis',(0.,0.,-1.));
#9741=DIRECTION('ref_axis',(1.,0.,0.));
#9742=DIRECTION('center_axis',(0.,0.,1.));
#9743=DIRECTION('ref_axis',(1.,0.,0.));
#9744=DIRECTION('center_axis',(0.,0.,1.));
#9745=DIRECTION('ref_axis',(1.,0.,0.));
#9746=DIRECTION('',(0.,0.,1.));
#9747=DIRECTION('center_axis',(0.,0.,-1.));
#9748=DIRECTION('ref_axis',(1.,0.,0.));
#9749=DIRECTION('center_axis',(0.,0.,1.));
#9750=DIRECTION('ref_axis',(1.,0.,0.));
#9751=DIRECTION('center_axis',(0.,0.,1.));
#9752=DIRECTION('ref_axis',(1.,0.,0.));
#9753=DIRECTION('',(0.,0.,1.));
#9754=DIRECTION('center_axis',(0.,0.,-1.));
#9755=DIRECTION('ref_axis',(1.,0.,0.));
#9756=DIRECTION('center_axis',(0.,0.,1.));
#9757=DIRECTION('ref_axis',(1.,0.,0.));
#9758=DIRECTION('center_axis',(0.,0.,1.));
#9759=DIRECTION('ref_axis',(1.,0.,0.));
#9760=DIRECTION('',(0.,0.,1.));
#9761=DIRECTION('center_axis',(0.,0.,-1.));
#9762=DIRECTION('ref_axis',(1.,0.,0.));
#9763=DIRECTION('center_axis',(0.,0.,1.));
#9764=DIRECTION('ref_axis',(1.,0.,0.));
#9765=DIRECTION('center_axis',(0.,0.,1.));
#9766=DIRECTION('ref_axis',(1.,0.,0.));
#9767=DIRECTION('',(0.,0.,1.));
#9768=DIRECTION('center_axis',(0.,0.,-1.));
#9769=DIRECTION('ref_axis',(1.,0.,0.));
#9770=DIRECTION('center_axis',(0.,0.,1.));
#9771=DIRECTION('ref_axis',(1.,0.,0.));
#9772=DIRECTION('center_axis',(0.,0.,1.));
#9773=DIRECTION('ref_axis',(1.,0.,0.));
#9774=DIRECTION('',(0.,0.,1.));
#9775=DIRECTION('center_axis',(0.,0.,-1.));
#9776=DIRECTION('ref_axis',(1.,0.,0.));
#9777=DIRECTION('center_axis',(0.,0.,1.));
#9778=DIRECTION('ref_axis',(1.,0.,0.));
#9779=DIRECTION('center_axis',(0.,0.,1.));
#9780=DIRECTION('ref_axis',(1.,0.,0.));
#9781=DIRECTION('',(0.,0.,1.));
#9782=DIRECTION('center_axis',(0.,0.,-1.));
#9783=DIRECTION('ref_axis',(1.,0.,0.));
#9784=DIRECTION('center_axis',(0.,0.,1.));
#9785=DIRECTION('ref_axis',(1.,0.,0.));
#9786=DIRECTION('center_axis',(0.,0.,1.));
#9787=DIRECTION('ref_axis',(1.,0.,0.));
#9788=DIRECTION('',(0.,0.,1.));
#9789=DIRECTION('center_axis',(0.,0.,-1.));
#9790=DIRECTION('ref_axis',(1.,0.,0.));
#9791=DIRECTION('center_axis',(0.,0.,1.));
#9792=DIRECTION('ref_axis',(1.,0.,0.));
#9793=DIRECTION('center_axis',(0.,0.,1.));
#9794=DIRECTION('ref_axis',(1.,0.,0.));
#9795=DIRECTION('',(0.,0.,1.));
#9796=DIRECTION('center_axis',(0.,0.,-1.));
#9797=DIRECTION('ref_axis',(1.,0.,0.));
#9798=DIRECTION('center_axis',(0.,0.,1.));
#9799=DIRECTION('ref_axis',(1.,0.,0.));
#9800=DIRECTION('center_axis',(0.,0.,1.));
#9801=DIRECTION('ref_axis',(1.,0.,0.));
#9802=DIRECTION('',(0.,0.,1.));
#9803=DIRECTION('center_axis',(0.,0.,-1.));
#9804=DIRECTION('ref_axis',(1.,0.,0.));
#9805=DIRECTION('center_axis',(0.,0.,1.));
#9806=DIRECTION('ref_axis',(1.,0.,0.));
#9807=DIRECTION('center_axis',(0.,0.,1.));
#9808=DIRECTION('ref_axis',(1.,0.,0.));
#9809=DIRECTION('',(0.,0.,1.));
#9810=DIRECTION('center_axis',(0.,0.,-1.));
#9811=DIRECTION('ref_axis',(1.,0.,0.));
#9812=DIRECTION('center_axis',(0.,0.,1.));
#9813=DIRECTION('ref_axis',(1.,0.,0.));
#9814=DIRECTION('center_axis',(0.,0.,1.));
#9815=DIRECTION('ref_axis',(1.,0.,0.));
#9816=DIRECTION('',(0.,0.,1.));
#9817=DIRECTION('center_axis',(0.,0.,-1.));
#9818=DIRECTION('ref_axis',(1.,0.,0.));
#9819=DIRECTION('center_axis',(0.,0.,1.));
#9820=DIRECTION('ref_axis',(1.,0.,0.));
#9821=DIRECTION('center_axis',(0.,0.,1.));
#9822=DIRECTION('ref_axis',(1.,0.,0.));
#9823=DIRECTION('',(0.,0.,1.));
#9824=DIRECTION('center_axis',(0.,0.,-1.));
#9825=DIRECTION('ref_axis',(1.,0.,0.));
#9826=DIRECTION('center_axis',(0.,0.,1.));
#9827=DIRECTION('ref_axis',(1.,0.,0.));
#9828=DIRECTION('center_axis',(0.,0.,1.));
#9829=DIRECTION('ref_axis',(1.,0.,0.));
#9830=DIRECTION('',(0.,0.,1.));
#9831=DIRECTION('center_axis',(0.,0.,-1.));
#9832=DIRECTION('ref_axis',(1.,0.,0.));
#9833=DIRECTION('center_axis',(0.,1.,0.));
#9834=DIRECTION('ref_axis',(-1.,0.,0.));
#9835=DIRECTION('',(-1.,0.,0.));
#9836=DIRECTION('',(0.,0.,1.));
#9837=DIRECTION('',(-1.,0.,0.));
#9838=DIRECTION('',(0.,0.,1.));
#9839=DIRECTION('center_axis',(1.,0.,0.));
#9840=DIRECTION('ref_axis',(0.,1.,0.));
#9841=DIRECTION('',(0.,1.,0.));
#9842=DIRECTION('',(0.,1.,0.));
#9843=DIRECTION('',(0.,0.,1.));
#9844=DIRECTION('center_axis',(0.,-1.,0.));
#9845=DIRECTION('ref_axis',(1.,0.,0.));
#9846=DIRECTION('',(1.,0.,0.));
#9847=DIRECTION('',(1.,0.,0.));
#9848=DIRECTION('',(0.,0.,1.));
#9849=DIRECTION('center_axis',(-1.,0.,0.));
#9850=DIRECTION('ref_axis',(0.,-1.,0.));
#9851=DIRECTION('',(0.,-1.,0.));
#9852=DIRECTION('',(0.,-1.,0.));
#9853=DIRECTION('center_axis',(0.,0.,1.));
#9854=DIRECTION('ref_axis',(1.,0.,0.));
#9855=DIRECTION('center_axis',(0.,0.,1.));
#9856=DIRECTION('ref_axis',(1.,0.,0.));
#11901=CARTESIAN_POINT('',(0.,0.,0.));
#11902=CARTESIAN_POINT('Origin',(19.5,12.5,5.1));
#11903=CARTESIAN_POINT('',(19.335,12.5,5.2));
#11904=CARTESIAN_POINT('Origin',(19.5,12.5,5.2));
#11905=CARTESIAN_POINT('',(19.335,12.5,6.4));
#11906=CARTESIAN_POINT('',(19.335,12.5,5.1));
#11907=CARTESIAN_POINT('Origin',(19.5,12.5,6.4));
#11908=CARTESIAN_POINT('Origin',(20.5,12.5,5.1));
#11909=CARTESIAN_POINT('',(20.335,12.5,5.2));
#11910=CARTESIAN_POINT('Origin',(20.5,12.5,5.2));
#11911=CARTESIAN_POINT('',(20.335,12.5,6.4));
#11912=CARTESIAN_POINT('',(20.335,12.5,5.1));
#11913=CARTESIAN_POINT('Origin',(20.5,12.5,6.4));
#11914=CARTESIAN_POINT('Origin',(20.,0.,5.1));
#11915=CARTESIAN_POINT('',(19.75,-3.06161699786838E-17,5.2));
#11916=CARTESIAN_POINT('Origin',(20.,0.,5.2));
#11917=CARTESIAN_POINT('',(19.75,3.06161699786838E-17,6.4));
#11918=CARTESIAN_POINT('',(19.75,-3.06161699786838E-17,5.1));
#11919=CARTESIAN_POINT('Origin',(20.,0.,6.4));
#11920=CARTESIAN_POINT('Origin',(25.5,8.1,5.1));
#11921=CARTESIAN_POINT('',(25.225,8.1,5.2));
#11922=CARTESIAN_POINT('Origin',(25.5,8.1,5.2));
#11923=CARTESIAN_POINT('',(25.225,8.1,6.4));
#11924=CARTESIAN_POINT('',(25.225,8.1,5.1));
#11925=CARTESIAN_POINT('Origin',(25.5,8.1,6.4));
#11926=CARTESIAN_POINT('Origin',(22.5,11.9,5.1));
#11927=CARTESIAN_POINT('',(22.225,11.9,5.2));
#11928=CARTESIAN_POINT('Origin',(22.5,11.9,5.2));
#11929=CARTESIAN_POINT('',(22.225,11.9,6.4));
#11930=CARTESIAN_POINT('',(22.225,11.9,5.1));
#11931=CARTESIAN_POINT('Origin',(22.5,11.9,6.4));
#11932=CARTESIAN_POINT('Origin',(22.5,8.1,5.1));
#11933=CARTESIAN_POINT('',(22.225,8.1,5.2));
#11934=CARTESIAN_POINT('Origin',(22.5,8.1,5.2));
#11935=CARTESIAN_POINT('',(22.225,8.1,6.4));
#11936=CARTESIAN_POINT('',(22.225,8.1,5.1));
#11937=CARTESIAN_POINT('Origin',(22.5,8.1,6.4));
#11938=CARTESIAN_POINT('Origin',(25.5,11.9,5.1));
#11939=CARTESIAN_POINT('',(25.225,11.9,5.2));
#11940=CARTESIAN_POINT('Origin',(25.5,11.9,5.2));
#11941=CARTESIAN_POINT('',(25.225,11.9,6.4));
#11942=CARTESIAN_POINT('',(25.225,11.9,5.1));
#11943=CARTESIAN_POINT('Origin',(25.5,11.9,6.4));
#11944=CARTESIAN_POINT('Origin',(17.5,8.1,5.1));
#11945=CARTESIAN_POINT('',(17.225,8.1,5.2));
#11946=CARTESIAN_POINT('Origin',(17.5,8.1,5.2));
#11947=CARTESIAN_POINT('',(17.225,8.1,6.4));
#11948=CARTESIAN_POINT('',(17.225,8.1,5.1));
#11949=CARTESIAN_POINT('Origin',(17.5,8.1,6.4));
#11950=CARTESIAN_POINT('Origin',(14.5,11.9,5.1));
#11951=CARTESIAN_POINT('',(14.225,11.9,5.2));
#11952=CARTESIAN_POINT('Origin',(14.5,11.9,5.2));
#11953=CARTESIAN_POINT('',(14.225,11.9,6.4));
#11954=CARTESIAN_POINT('',(14.225,11.9,5.1));
#11955=CARTESIAN_POINT('Origin',(14.5,11.9,6.4));
#11956=CARTESIAN_POINT('Origin',(14.5,8.1,5.1));
#11957=CARTESIAN_POINT('',(14.225,8.1,5.2));
#11958=CARTESIAN_POINT('Origin',(14.5,8.1,5.2));
#11959=CARTESIAN_POINT('',(14.225,8.1,6.4));
#11960=CARTESIAN_POINT('',(14.225,8.1,5.1));
#11961=CARTESIAN_POINT('Origin',(14.5,8.1,6.4));
#11962=CARTESIAN_POINT('Origin',(17.5,11.9,5.1));
#11963=CARTESIAN_POINT('',(17.225,11.9,5.2));
#11964=CARTESIAN_POINT('Origin',(17.5,11.9,5.2));
#11965=CARTESIAN_POINT('',(17.225,11.9,6.4));
#11966=CARTESIAN_POINT('',(17.225,11.9,5.1));
#11967=CARTESIAN_POINT('Origin',(17.5,11.9,6.4));
#11968=CARTESIAN_POINT('Origin',(25.5,-11.9,5.1));
#11969=CARTESIAN_POINT('',(25.225,-11.9,5.2));
#11970=CARTESIAN_POINT('Origin',(25.5,-11.9,5.2));
#11971=CARTESIAN_POINT('',(25.225,-11.9,6.4));
#11972=CARTESIAN_POINT('',(25.225,-11.9,5.1));
#11973=CARTESIAN_POINT('Origin',(25.5,-11.9,6.4));
#11974=CARTESIAN_POINT('Origin',(22.5,-8.1,5.1));
#11975=CARTESIAN_POINT('',(22.225,-8.1,5.2));
#11976=CARTESIAN_POINT('Origin',(22.5,-8.1,5.2));
#11977=CARTESIAN_POINT('',(22.225,-8.1,6.4));
#11978=CARTESIAN_POINT('',(22.225,-8.1,5.1));
#11979=CARTESIAN_POINT('Origin',(22.5,-8.1,6.4));
#11980=CARTESIAN_POINT('Origin',(22.5,-11.9,5.1));
#11981=CARTESIAN_POINT('',(22.225,-11.9,5.2));
#11982=CARTESIAN_POINT('Origin',(22.5,-11.9,5.2));
#11983=CARTESIAN_POINT('',(22.225,-11.9,6.4));
#11984=CARTESIAN_POINT('',(22.225,-11.9,5.1));
#11985=CARTESIAN_POINT('Origin',(22.5,-11.9,6.4));
#11986=CARTESIAN_POINT('Origin',(25.5,-8.1,5.1));
#11987=CARTESIAN_POINT('',(25.225,-8.1,5.2));
#11988=CARTESIAN_POINT('Origin',(25.5,-8.1,5.2));
#11989=CARTESIAN_POINT('',(25.225,-8.1,6.4));
#11990=CARTESIAN_POINT('',(25.225,-8.1,5.1));
#11991=CARTESIAN_POINT('Origin',(25.5,-8.1,6.4));
#11992=CARTESIAN_POINT('Origin',(17.5,-11.9,5.1));
#11993=CARTESIAN_POINT('',(17.225,-11.9,5.2));
#11994=CARTESIAN_POINT('Origin',(17.5,-11.9,5.2));
#11995=CARTESIAN_POINT('',(17.225,-11.9,6.4));
#11996=CARTESIAN_POINT('',(17.225,-11.9,5.1));
#11997=CARTESIAN_POINT('Origin',(17.5,-11.9,6.4));
#11998=CARTESIAN_POINT('Origin',(14.5,-8.1,5.1));
#11999=CARTESIAN_POINT('',(14.225,-8.1,5.2));
#12000=CARTESIAN_POINT('Origin',(14.5,-8.1,5.2));
#12001=CARTESIAN_POINT('',(14.225,-8.1,6.4));
#12002=CARTESIAN_POINT('',(14.225,-8.1,5.1));
#12003=CARTESIAN_POINT('Origin',(14.5,-8.1,6.4));
#12004=CARTESIAN_POINT('Origin',(14.5,-11.9,5.1));
#12005=CARTESIAN_POINT('',(14.225,-11.9,5.2));
#12006=CARTESIAN_POINT('Origin',(14.5,-11.9,5.2));
#12007=CARTESIAN_POINT('',(14.225,-11.9,6.4));
#12008=CARTESIAN_POINT('',(14.225,-11.9,5.1));
#12009=CARTESIAN_POINT('Origin',(14.5,-11.9,6.4));
#12010=CARTESIAN_POINT('Origin',(17.5,-8.1,5.1));
#12011=CARTESIAN_POINT('',(17.225,-8.1,5.2));
#12012=CARTESIAN_POINT('Origin',(17.5,-8.1,5.2));
#12013=CARTESIAN_POINT('',(17.225,-8.1,6.4));
#12014=CARTESIAN_POINT('',(17.225,-8.1,5.1));
#12015=CARTESIAN_POINT('Origin',(17.5,-8.1,6.4));
#12016=CARTESIAN_POINT('Origin',(28.,13.,5.2));
#12017=CARTESIAN_POINT('',(28.,13.,5.2));
#12018=CARTESIAN_POINT('',(12.,13.,5.2));
#12019=CARTESIAN_POINT('',(28.,13.,5.2));
#12020=CARTESIAN_POINT('',(12.,13.,6.4));
#12021=CARTESIAN_POINT('',(12.,13.,5.2));
#12022=CARTESIAN_POINT('',(28.,13.,6.4));
#12023=CARTESIAN_POINT('',(28.,13.,6.4));
#12024=CARTESIAN_POINT('',(28.,13.,5.2));
#12025=CARTESIAN_POINT('Origin',(28.,-13.,5.2));
#12026=CARTESIAN_POINT('',(28.,-13.,5.2));
#12027=CARTESIAN_POINT('',(28.,-13.,5.2));
#12028=CARTESIAN_POINT('',(28.,-13.,6.4));
#12029=CARTESIAN_POINT('',(28.,-13.,6.4));
#12030=CARTESIAN_POINT('',(28.,-13.,5.2));
#12031=CARTESIAN_POINT('Origin',(12.,-13.,5.2));
#12032=CARTESIAN_POINT('',(12.,-13.,5.2));
#12033=CARTESIAN_POINT('',(12.,-13.,5.2));
#12034=CARTESIAN_POINT('',(12.,-13.,6.4));
#12035=CARTESIAN_POINT('',(12.,-13.,6.4));
#12036=CARTESIAN_POINT('',(12.,-13.,5.2));
#12037=CARTESIAN_POINT('Origin',(12.,13.,5.2));
#12038=CARTESIAN_POINT('',(12.,13.,5.2));
#12039=CARTESIAN_POINT('',(12.,13.,6.4));
#12040=CARTESIAN_POINT('Origin',(20.,0.,6.4));
#12041=CARTESIAN_POINT('Origin',(20.,0.,5.2));
#12755=UNCERTAINTY_MEASURE_WITH_UNIT(LENGTH_MEASURE(0.001),#12805,
'DISTANCE_ACCURACY_VALUE',
'Maximum model space distance between geometric entities at asserted c
onnectivities');
#12768=UNCERTAINTY_MEASURE_WITH_UNIT(LENGTH_MEASURE(0.001),#12805,
'DISTANCE_ACCURACY_VALUE',
'Maximum model space distance between geometric entities at asserted c
onnectivities');
#12791=(
GEOMETRIC_REPRESENTATION_CONTEXT(3)
GLOBAL_UNCERTAINTY_ASSIGNED_CONTEXT((#12755))
GLOBAL_UNIT_ASSIGNED_CONTEXT((#12805,#12807,#12808))
REPRESENTATION_CONTEXT('','3D')
);
#12804=(
GEOMETRIC_REPRESENTATION_CONTEXT(3)
GLOBAL_UNCERTAINTY_ASSIGNED_CONTEXT((#12768))
GLOBAL_UNIT_ASSIGNED_CONTEXT((#12805,#12807,#12808))
REPRESENTATION_CONTEXT('','3D')
);
#12805=(
LENGTH_UNIT()
NAMED_UNIT(*)
SI_UNIT(.CENTI.,.METRE.)
);
#12807=(
NAMED_UNIT(*)
PLANE_ANGLE_UNIT()
SI_UNIT($,.RADIAN.)
);
#12808=(
NAMED_UNIT(*)
SI_UNIT($,.STERADIAN.)
SOLID_ANGLE_UNIT()
);
#12831=SHAPE_DEFINITION_REPRESENTATION(#12866,#13021);
#12866=PRODUCT_DEFINITION_SHAPE('',$,#13057);
#13021=SHAPE_REPRESENTATION('',(#8110),#12791);
#13034=PRODUCT_DEFINITION_CONTEXT('part definition',#13141,'design');
#13057=PRODUCT_DEFINITION('Bridge table','Bridge table',#13092,#13034);
#13092=PRODUCT_DEFINITION_FORMATION('',$,#13165);
#13141=APPLICATION_CONTEXT(
'Core Data for Automotive Mechanical Design Process');
#13142=PRODUCT_CONTEXT('part definition',#13141,'mechanical');
#13165=PRODUCT('Bridge table','Bridge table','Bridge table',(#13142));
#13227=COLOUR_RGB('Light Blue',0.38,0.62,0.78);
#13228=FILL_AREA_STYLE_COLOUR('',#13227);
#13229=FILL_AREA_STYLE('',(#13228));
#13230=SURFACE_STYLE_FILL_AREA(#13229);
#13231=SURFACE_SIDE_STYLE('',(#13230));
#13232=SURFACE_STYLE_USAGE(.BOTH.,#13231);
#13233=PRESENTATION_STYLE_ASSIGNMENT((#13232));
ENDSEC;
END-ISO-10303-21;
